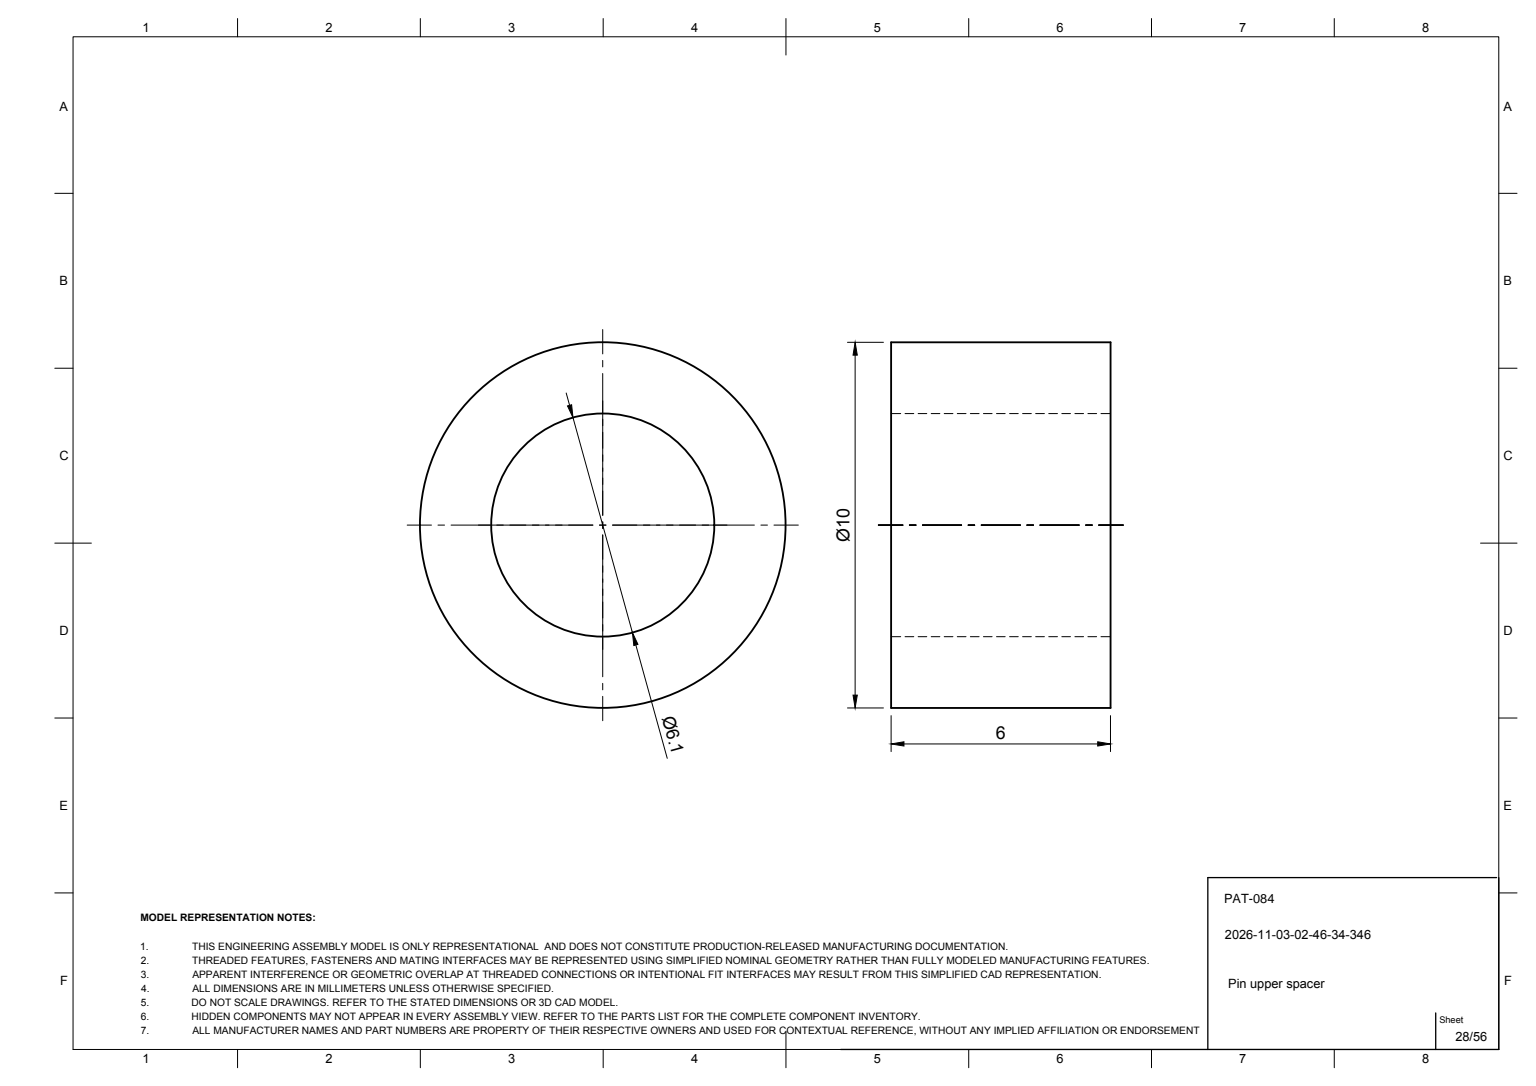
ISO-10303-21;
HEADER;
/* Generated by software containing ST-Developer
 * from STEP Tools, Inc. (www.steptools.com) 
 */

FILE_DESCRIPTION(
/* description */ ('Quick-return (Whitworth) mechanism'),
/* implementation_level */ '2;1');

FILE_NAME(
/* name */ 'Pin upper spacer.step',
/* time_stamp */ '2026-10-28T03:25:57-07:00',
/* author */ (''),
/* organization */ (''),
/* preprocessor_version */ 'ST-DEVELOPER v20.2',
/* originating_system */ 'Autodesk Translation Framework v15.17.0.0',
/* authorisation */ '');

FILE_SCHEMA (('AUTOMOTIVE_DESIGN { 1 0 10303 214 3 1 1 }'));
ENDSEC;

DATA;
#10=MECHANICAL_DESIGN_GEOMETRIC_PRESENTATION_REPRESENTATION('',(#517),#14878);
#421=SHAPE_REPRESENTATION_RELATIONSHIP('SRR','None',#15091,#465);
#465=ADVANCED_BREP_SHAPE_REPRESENTATION('',(#569),#14848);
#517=STYLED_ITEM('',(#15406),#569);
#569=MANIFOLD_SOLID_BREP('Body1',#7871);
#720=FACE_BOUND('',#1891,.T.);
#721=FACE_BOUND('',#1893,.T.);
#897=PLANE('',#8943);
#898=PLANE('',#8944);
#1293=FACE_OUTER_BOUND('',#1888,.T.);
#1294=FACE_OUTER_BOUND('',#1889,.T.);
#1295=FACE_OUTER_BOUND('',#1890,.T.);
#1296=FACE_OUTER_BOUND('',#1892,.T.);
#1888=EDGE_LOOP('',(#6294,#6295,#6296,#6297));
#1889=EDGE_LOOP('',(#6298,#6299,#6300,#6301));
#1890=EDGE_LOOP('',(#6302));
#1891=EDGE_LOOP('',(#6303));
#1892=EDGE_LOOP('',(#6304));
#1893=EDGE_LOOP('',(#6305));
#2377=LINE('',#13631,#2900);
#2378=LINE('',#13637,#2901);
#2900=VECTOR('',#10714,0.305);
#2901=VECTOR('',#10721,0.5);
#3494=CIRCLE('',#8938,0.305);
#3495=CIRCLE('',#8939,0.305);
#3496=CIRCLE('',#8941,0.5);
#3497=CIRCLE('',#8942,0.5);
#3986=VERTEX_POINT('',#13628);
#3987=VERTEX_POINT('',#13630);
#3988=VERTEX_POINT('',#13634);
#3989=VERTEX_POINT('',#13636);
#4804=EDGE_CURVE('',#3986,#3986,#3494,.T.);
#4805=EDGE_CURVE('',#3986,#3987,#2377,.T.);
#4806=EDGE_CURVE('',#3987,#3987,#3495,.T.);
#4807=EDGE_CURVE('',#3988,#3988,#3496,.T.);
#4808=EDGE_CURVE('',#3988,#3989,#2378,.T.);
#4809=EDGE_CURVE('',#3989,#3989,#3497,.T.);
#6294=ORIENTED_EDGE('',*,*,#4804,.F.);
#6295=ORIENTED_EDGE('',*,*,#4805,.T.);
#6296=ORIENTED_EDGE('',*,*,#4806,.T.);
#6297=ORIENTED_EDGE('',*,*,#4805,.F.);
#6298=ORIENTED_EDGE('',*,*,#4807,.F.);
#6299=ORIENTED_EDGE('',*,*,#4808,.T.);
#6300=ORIENTED_EDGE('',*,*,#4809,.T.);
#6301=ORIENTED_EDGE('',*,*,#4808,.F.);
#6302=ORIENTED_EDGE('',*,*,#4807,.T.);
#6303=ORIENTED_EDGE('',*,*,#4804,.T.);
#6304=ORIENTED_EDGE('',*,*,#4809,.F.);
#6305=ORIENTED_EDGE('',*,*,#4806,.F.);
#7319=CYLINDRICAL_SURFACE('',#8937,0.305);
#7320=CYLINDRICAL_SURFACE('',#8940,0.5);
#7624=ADVANCED_FACE('',(#1293),#7319,.F.);
#7625=ADVANCED_FACE('',(#1294),#7320,.T.);
#7626=ADVANCED_FACE('',(#1295,#720),#897,.T.);
#7627=ADVANCED_FACE('',(#1296,#721),#898,.F.);
#7871=CLOSED_SHELL('',(#7624,#7625,#7626,#7627));
#8936=AXIS2_PLACEMENT_3D('',#13626,#10708,#10709);
#8937=AXIS2_PLACEMENT_3D('',#13627,#10710,#10711);
#8938=AXIS2_PLACEMENT_3D('',#13629,#10712,#10713);
#8939=AXIS2_PLACEMENT_3D('',#13632,#10715,#10716);
#8940=AXIS2_PLACEMENT_3D('',#13633,#10717,#10718);
#8941=AXIS2_PLACEMENT_3D('',#13635,#10719,#10720);
#8942=AXIS2_PLACEMENT_3D('',#13638,#10722,#10723);
#8943=AXIS2_PLACEMENT_3D('',#13639,#10724,#10725);
#8944=AXIS2_PLACEMENT_3D('',#13640,#10726,#10727);
#10708=DIRECTION('axis',(0.,0.,1.));
#10709=DIRECTION('refdir',(1.,0.,0.));
#10710=DIRECTION('center_axis',(0.,0.,1.));
#10711=DIRECTION('ref_axis',(1.,0.,0.));
#10712=DIRECTION('center_axis',(0.,0.,-1.));
#10713=DIRECTION('ref_axis',(1.,0.,0.));
#10714=DIRECTION('',(0.,0.,-1.));
#10715=DIRECTION('center_axis',(0.,0.,-1.));
#10716=DIRECTION('ref_axis',(1.,0.,0.));
#10717=DIRECTION('center_axis',(0.,0.,1.));
#10718=DIRECTION('ref_axis',(1.,0.,0.));
#10719=DIRECTION('center_axis',(0.,0.,1.));
#10720=DIRECTION('ref_axis',(1.,0.,0.));
#10721=DIRECTION('',(0.,0.,-1.));
#10722=DIRECTION('center_axis',(0.,0.,1.));
#10723=DIRECTION('ref_axis',(1.,0.,0.));
#10724=DIRECTION('center_axis',(0.,0.,1.));
#10725=DIRECTION('ref_axis',(1.,0.,0.));
#10726=DIRECTION('center_axis',(0.,0.,1.));
#10727=DIRECTION('ref_axis',(1.,0.,0.));
#13626=CARTESIAN_POINT('',(0.,0.,0.));
#13627=CARTESIAN_POINT('Origin',(0.,9.,7.4));
#13628=CARTESIAN_POINT('',(-0.305,9.,8.));
#13629=CARTESIAN_POINT('Origin',(0.,9.,8.));
#13630=CARTESIAN_POINT('',(-0.305,9.,7.4));
#13631=CARTESIAN_POINT('',(-0.305,9.,7.4));
#13632=CARTESIAN_POINT('Origin',(0.,9.,7.4));
#13633=CARTESIAN_POINT('Origin',(0.,9.,7.4));
#13634=CARTESIAN_POINT('',(-0.5,9.,8.));
#13635=CARTESIAN_POINT('Origin',(0.,9.,8.));
#13636=CARTESIAN_POINT('',(-0.5,9.,7.4));
#13637=CARTESIAN_POINT('',(-0.5,9.,7.4));
#13638=CARTESIAN_POINT('Origin',(0.,9.,7.4));
#13639=CARTESIAN_POINT('Origin',(0.,9.,8.));
#13640=CARTESIAN_POINT('Origin',(0.,9.,7.4));
#14794=UNCERTAINTY_MEASURE_WITH_UNIT(LENGTH_MEASURE(0.001),#14879,
'DISTANCE_ACCURACY_VALUE',
'Maximum model space distance between geometric entities at asserted c
onnectivities');
#14824=UNCERTAINTY_MEASURE_WITH_UNIT(LENGTH_MEASURE(0.001),#14879,
'DISTANCE_ACCURACY_VALUE',
'Maximum model space distance between geometric entities at asserted c
onnectivities');
#14848=(
GEOMETRIC_REPRESENTATION_CONTEXT(3)
GLOBAL_UNCERTAINTY_ASSIGNED_CONTEXT((#14794))
GLOBAL_UNIT_ASSIGNED_CONTEXT((#14879,#14881,#14882))
REPRESENTATION_CONTEXT('','3D')
);
#14878=(
GEOMETRIC_REPRESENTATION_CONTEXT(3)
GLOBAL_UNCERTAINTY_ASSIGNED_CONTEXT((#14824))
GLOBAL_UNIT_ASSIGNED_CONTEXT((#14879,#14881,#14882))
REPRESENTATION_CONTEXT('','3D')
);
#14879=(
LENGTH_UNIT()
NAMED_UNIT(*)
SI_UNIT(.CENTI.,.METRE.)
);
#14881=(
NAMED_UNIT(*)
PLANE_ANGLE_UNIT()
SI_UNIT($,.RADIAN.)
);
#14882=(
NAMED_UNIT(*)
SI_UNIT($,.STERADIAN.)
SOLID_ANGLE_UNIT()
);
#14906=SHAPE_DEFINITION_REPRESENTATION(#14964,#15091);
#14964=PRODUCT_DEFINITION_SHAPE('',$,#15145);
#15091=SHAPE_REPRESENTATION('',(#8936),#14848);
#15121=PRODUCT_DEFINITION_CONTEXT('part definition',#15282,'design');
#15145=PRODUCT_DEFINITION('Pin upper spacer','Pin upper spacer',#15198,
#15121);
#15198=PRODUCT_DEFINITION_FORMATION('',$,#15307);
#15282=APPLICATION_CONTEXT(
'Core Data for Automotive Mechanical Design Process');
#15283=PRODUCT_CONTEXT('part definition',#15282,'mechanical');
#15307=PRODUCT('Pin upper spacer','Pin upper spacer','Pin upper spacer',
(#15283));
#15400=COLOUR_RGB('Grey',0.48,0.52,0.57);
#15401=FILL_AREA_STYLE_COLOUR('',#15400);
#15402=FILL_AREA_STYLE('',(#15401));
#15403=SURFACE_STYLE_FILL_AREA(#15402);
#15404=SURFACE_SIDE_STYLE('',(#15403));
#15405=SURFACE_STYLE_USAGE(.BOTH.,#15404);
#15406=PRESENTATION_STYLE_ASSIGNMENT((#15405));
ENDSEC;
END-ISO-10303-21;
